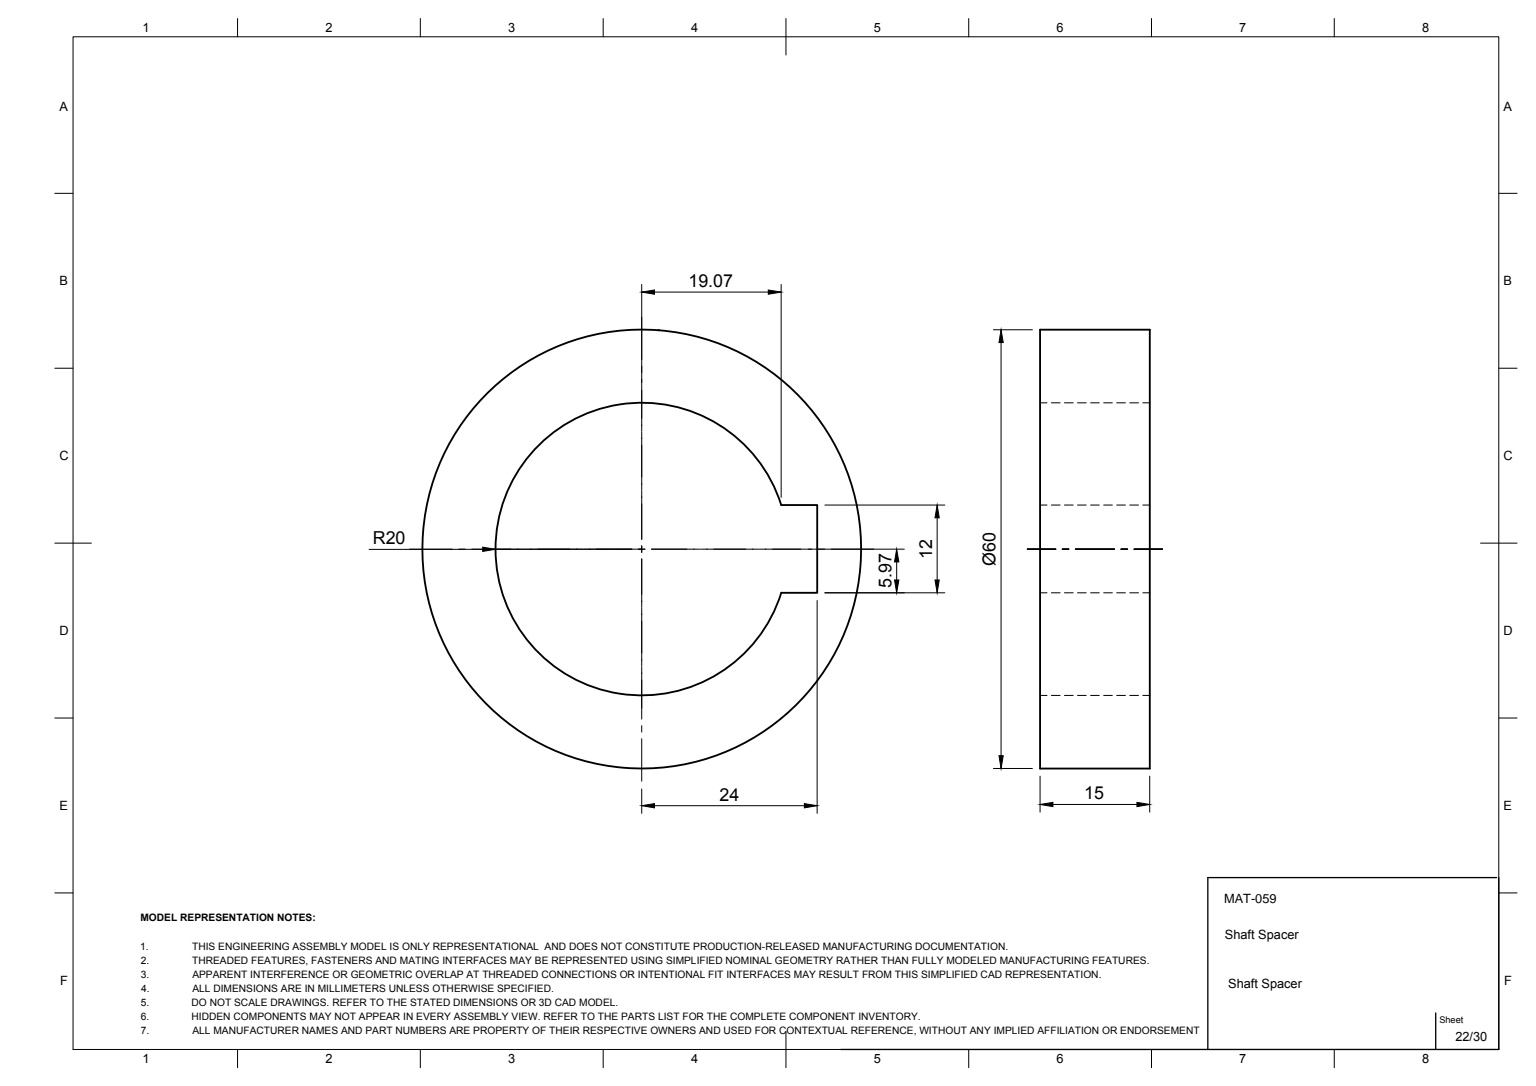
ISO-10303-21;
HEADER;
/* Generated by software containing ST-Developer
 * from STEP Tools, Inc. (www.steptools.com) 
 */

FILE_DESCRIPTION(
/* description */ ('', 'CAx-IF Rec.Pracs.---Representation and Presentation of Product Manufa
cturing Information (PMI)---4.0---2014-10-13'),
/* implementation_level */ '2;1');

FILE_NAME(
/* name */ 'Shaft Spacer.step',
/* time_stamp */ '2026-10-28T23:00:48+01:00',
/* author */ (''),
/* organization */ (''),
/* preprocessor_version */ 'ST-DEVELOPER v20.2',
/* originating_system */ 'Autodesk Translation Framework v15.17.0.0',
/* authorisation */ '');

FILE_SCHEMA (('AP242_MANAGED_MODEL_BASED_3D_ENGINEERING_MIM_LF { 1 0 10303 442 2 1 4 }'));
ENDSEC;

DATA;
#10=MECHANICAL_DESIGN_GEOMETRIC_PRESENTATION_REPRESENTATION('',(#994),#61811);
#930=SHAPE_REPRESENTATION_RELATIONSHIP('SRR','None',#61990,#955);
#955=ADVANCED_BREP_SHAPE_REPRESENTATION('',(#1033),#61803);
#994=STYLED_ITEM('',(#62156),#1033);
#1033=MANIFOLD_SOLID_BREP('Body1',#33824);
#1391=CYLINDRICAL_SURFACE('',#36117,20.);
#1392=CYLINDRICAL_SURFACE('',#36119,30.);
#2127=FACE_BOUND('',#7392,.T.);
#2128=FACE_BOUND('',#7396,.T.);
#3117=CIRCLE('',#36115,30.);
#3118=CIRCLE('',#36116,20.);
#3119=CIRCLE('',#36118,20.);
#3120=CIRCLE('',#36120,30.);
#5261=FACE_OUTER_BOUND('',#7388,.T.);
#5262=FACE_OUTER_BOUND('',#7389,.T.);
#5263=FACE_OUTER_BOUND('',#7390,.T.);
#5264=FACE_OUTER_BOUND('',#7391,.T.);
#5265=FACE_OUTER_BOUND('',#7393,.T.);
#5266=FACE_OUTER_BOUND('',#7394,.T.);
#5267=FACE_OUTER_BOUND('',#7395,.T.);
#7388=EDGE_LOOP('',(#26536,#26537,#26538,#26539));
#7389=EDGE_LOOP('',(#26540,#26541,#26542,#26543));
#7390=EDGE_LOOP('',(#26544,#26545,#26546,#26547));
#7391=EDGE_LOOP('',(#26548));
#7392=EDGE_LOOP('',(#26549,#26550,#26551,#26552));
#7393=EDGE_LOOP('',(#26553,#26554,#26555,#26556));
#7394=EDGE_LOOP('',(#26557,#26558,#26559,#26560));
#7395=EDGE_LOOP('',(#26561));
#7396=EDGE_LOOP('',(#26562,#26563,#26564,#26565));
#9813=LINE('',#56343,#12360);
#9814=LINE('',#56345,#12361);
#9815=LINE('',#56347,#12362);
#9816=LINE('',#56348,#12363);
#9817=LINE('',#56351,#12364);
#9818=LINE('',#56353,#12365);
#9819=LINE('',#56354,#12366);
#9820=LINE('',#56358,#12367);
#9821=LINE('',#56359,#12368);
#9822=LINE('',#56360,#12369);
#9823=LINE('',#56370,#12370);
#12360=VECTOR('',#43633,10.);
#12361=VECTOR('',#43634,10.);
#12362=VECTOR('',#43635,10.);
#12363=VECTOR('',#43636,10.);
#12364=VECTOR('',#43639,10.);
#12365=VECTOR('',#43640,10.);
#12366=VECTOR('',#43641,10.);
#12367=VECTOR('',#43644,10.);
#12368=VECTOR('',#43645,10.);
#12369=VECTOR('',#43646,10.);
#12370=VECTOR('',#43661,30.);
#15097=VERTEX_POINT('',#56341);
#15098=VERTEX_POINT('',#56342);
#15099=VERTEX_POINT('',#56344);
#15100=VERTEX_POINT('',#56346);
#15101=VERTEX_POINT('',#56350);
#15102=VERTEX_POINT('',#56352);
#15103=VERTEX_POINT('',#56356);
#15104=VERTEX_POINT('',#56357);
#15105=VERTEX_POINT('',#56362);
#15106=VERTEX_POINT('',#56368);
#19170=EDGE_CURVE('',#15097,#15098,#9813,.T.);
#19171=EDGE_CURVE('',#15099,#15097,#9814,.T.);
#19172=EDGE_CURVE('',#15099,#15100,#9815,.T.);
#19173=EDGE_CURVE('',#15098,#15100,#9816,.T.);
#19174=EDGE_CURVE('',#15101,#15099,#9817,.T.);
#19175=EDGE_CURVE('',#15101,#15102,#9818,.T.);
#19176=EDGE_CURVE('',#15100,#15102,#9819,.T.);
#19177=EDGE_CURVE('',#15103,#15104,#9820,.T.);
#19178=EDGE_CURVE('',#15102,#15103,#9821,.T.);
#19179=EDGE_CURVE('',#15104,#15101,#9822,.T.);
#19180=EDGE_CURVE('',#15105,#15105,#3117,.T.);
#19181=EDGE_CURVE('',#15103,#15098,#3118,.T.);
#19182=EDGE_CURVE('',#15097,#15104,#3119,.T.);
#19183=EDGE_CURVE('',#15106,#15106,#3120,.T.);
#19184=EDGE_CURVE('',#15106,#15105,#9823,.T.);
#26536=ORIENTED_EDGE('',*,*,#19170,.F.);
#26537=ORIENTED_EDGE('',*,*,#19171,.F.);
#26538=ORIENTED_EDGE('',*,*,#19172,.T.);
#26539=ORIENTED_EDGE('',*,*,#19173,.F.);
#26540=ORIENTED_EDGE('',*,*,#19174,.F.);
#26541=ORIENTED_EDGE('',*,*,#19175,.T.);
#26542=ORIENTED_EDGE('',*,*,#19176,.F.);
#26543=ORIENTED_EDGE('',*,*,#19172,.F.);
#26544=ORIENTED_EDGE('',*,*,#19177,.F.);
#26545=ORIENTED_EDGE('',*,*,#19178,.F.);
#26546=ORIENTED_EDGE('',*,*,#19175,.F.);
#26547=ORIENTED_EDGE('',*,*,#19179,.F.);
#26548=ORIENTED_EDGE('',*,*,#19180,.T.);
#26549=ORIENTED_EDGE('',*,*,#19173,.T.);
#26550=ORIENTED_EDGE('',*,*,#19176,.T.);
#26551=ORIENTED_EDGE('',*,*,#19178,.T.);
#26552=ORIENTED_EDGE('',*,*,#19181,.T.);
#26553=ORIENTED_EDGE('',*,*,#19170,.T.);
#26554=ORIENTED_EDGE('',*,*,#19181,.F.);
#26555=ORIENTED_EDGE('',*,*,#19177,.T.);
#26556=ORIENTED_EDGE('',*,*,#19182,.F.);
#26557=ORIENTED_EDGE('',*,*,#19183,.F.);
#26558=ORIENTED_EDGE('',*,*,#19184,.T.);
#26559=ORIENTED_EDGE('',*,*,#19180,.F.);
#26560=ORIENTED_EDGE('',*,*,#19184,.F.);
#26561=ORIENTED_EDGE('',*,*,#19183,.T.);
#26562=ORIENTED_EDGE('',*,*,#19171,.T.);
#26563=ORIENTED_EDGE('',*,*,#19182,.T.);
#26564=ORIENTED_EDGE('',*,*,#19179,.T.);
#26565=ORIENTED_EDGE('',*,*,#19174,.T.);
#31650=PLANE('',#36111);
#31651=PLANE('',#36112);
#31652=PLANE('',#36113);
#31653=PLANE('',#36114);
#31654=PLANE('',#36121);
#32942=ADVANCED_FACE('',(#5261),#31650,.F.);
#32943=ADVANCED_FACE('',(#5262),#31651,.F.);
#32944=ADVANCED_FACE('',(#5263),#31652,.F.);
#32945=ADVANCED_FACE('',(#5264,#2127),#31653,.T.);
#32946=ADVANCED_FACE('',(#5265),#1391,.F.);
#32947=ADVANCED_FACE('',(#5266),#1392,.T.);
#32948=ADVANCED_FACE('',(#5267,#2128),#31654,.F.);
#33824=CLOSED_SHELL('',(#32942,#32943,#32944,#32945,#32946,#32947,#32948));
#36110=AXIS2_PLACEMENT_3D('',#56339,#43629,#43630);
#36111=AXIS2_PLACEMENT_3D('',#56340,#43631,#43632);
#36112=AXIS2_PLACEMENT_3D('',#56349,#43637,#43638);
#36113=AXIS2_PLACEMENT_3D('',#56355,#43642,#43643);
#36114=AXIS2_PLACEMENT_3D('',#56361,#43647,#43648);
#36115=AXIS2_PLACEMENT_3D('',#56363,#43649,#43650);
#36116=AXIS2_PLACEMENT_3D('',#56364,#43651,#43652);
#36117=AXIS2_PLACEMENT_3D('',#56365,#43653,#43654);
#36118=AXIS2_PLACEMENT_3D('',#56366,#43655,#43656);
#36119=AXIS2_PLACEMENT_3D('',#56367,#43657,#43658);
#36120=AXIS2_PLACEMENT_3D('',#56369,#43659,#43660);
#36121=AXIS2_PLACEMENT_3D('',#56371,#43662,#43663);
#43629=DIRECTION('axis',(0.,0.,1.));
#43630=DIRECTION('refdir',(1.,0.,0.));
#43631=DIRECTION('center_axis',(-0.996957691137886,1.38453029710175E-15,
-0.0779446090567869));
#43632=DIRECTION('ref_axis',(-0.0779446090567869,-2.95972462712666E-15,
0.996957691137886));
#43633=DIRECTION('',(1.14962354933188E-15,1.,3.05863690339901E-15));
#43634=DIRECTION('',(-0.0779446090567869,-2.95972462712666E-15,0.996957691137886));
#43635=DIRECTION('',(1.14962354933188E-15,1.,3.05863690339901E-15));
#43636=DIRECTION('',(0.0779446090567869,2.95972462712666E-15,-0.996957691137886));
#43637=DIRECTION('center_axis',(0.0779446090567869,2.95972462712666E-15,
-0.996957691137886));
#43638=DIRECTION('ref_axis',(-0.996957691137886,1.38453029710175E-15,-0.0779446090567869));
#43639=DIRECTION('',(-0.996957691137886,1.38453029710175E-15,-0.0779446090567869));
#43640=DIRECTION('',(1.14962354933188E-15,1.,3.05863690339901E-15));
#43641=DIRECTION('',(0.996957691137886,-1.38453029710175E-15,0.0779446090567869));
#43642=DIRECTION('center_axis',(0.996957691137886,-1.38453029710175E-15,
0.0779446090567869));
#43643=DIRECTION('ref_axis',(0.0779446090567869,2.95972462712666E-15,-0.996957691137886));
#43644=DIRECTION('',(-1.14962354933188E-15,-1.,-3.05863690339901E-15));
#43645=DIRECTION('',(-0.0779446090567869,-2.95972462712666E-15,0.996957691137886));
#43646=DIRECTION('',(0.0779446090567869,2.95972462712666E-15,-0.996957691137886));
#43647=DIRECTION('center_axis',(1.14962354933188E-15,1.,3.05863690339901E-15));
#43648=DIRECTION('ref_axis',(0.996957691137886,-1.38453029710175E-15,0.0779446090567869));
#43649=DIRECTION('center_axis',(1.14962354933188E-15,1.,3.05863690339901E-15));
#43650=DIRECTION('ref_axis',(0.996957691137886,-1.38453029710175E-15,0.077944609056787));
#43651=DIRECTION('center_axis',(-1.14962354933188E-15,-1.,-3.05863690339901E-15));
#43652=DIRECTION('ref_axis',(0.996957691137886,-1.38453029710175E-15,0.077944609056787));
#43653=DIRECTION('center_axis',(-1.14962354933188E-15,-1.,-3.05863690339901E-15));
#43654=DIRECTION('ref_axis',(-0.079454779543177,-2.95762384959718E-15,0.99683847137224));
#43655=DIRECTION('center_axis',(1.14962354933188E-15,1.,3.05863690339901E-15));
#43656=DIRECTION('ref_axis',(0.996957691137886,-1.38453029710175E-15,0.077944609056787));
#43657=DIRECTION('center_axis',(-1.14962354933188E-15,-1.,-3.05863690339901E-15));
#43658=DIRECTION('ref_axis',(0.996957691137886,-1.38453029710175E-15,0.077944609056787));
#43659=DIRECTION('center_axis',(-1.14962354933188E-15,-1.,-3.05863690339901E-15));
#43660=DIRECTION('ref_axis',(0.996957691137886,-1.38453029710175E-15,0.077944609056787));
#43661=DIRECTION('',(1.14962354933188E-15,1.,3.05863690339901E-15));
#43662=DIRECTION('center_axis',(1.14962354933188E-15,1.,3.05863690339901E-15));
#43663=DIRECTION('ref_axis',(0.996957691137886,-1.38453029710175E-15,0.0779446090567869));
#56339=CARTESIAN_POINT('',(0.,0.,0.));
#56340=CARTESIAN_POINT('Origin',(371.018259814925,-255.47200726879,420.650814731371));
#56341=CARTESIAN_POINT('',(370.635385768447,-255.47200726879,425.548000437897));
#56342=CARTESIAN_POINT('',(370.635385768447,-240.47200726879,425.548000437897));
#56343=CARTESIAN_POINT('',(370.635385768447,-240.47200726879,425.548000437897));
#56344=CARTESIAN_POINT('',(371.018259814925,-255.47200726879,420.650814731371));
#56345=CARTESIAN_POINT('',(370.082925320099,-255.47200726879,432.614296615326));
#56346=CARTESIAN_POINT('',(371.018259814925,-240.47200726879,420.650814731371));
#56347=CARTESIAN_POINT('',(371.018259814925,-255.47200726879,420.650814731371));
#56348=CARTESIAN_POINT('',(370.082925320099,-240.47200726879,432.614296615326));
#56349=CARTESIAN_POINT('Origin',(382.98175210858,-255.47200726879,421.586150040052));
#56350=CARTESIAN_POINT('',(382.98175210858,-255.47200726879,421.586150040052));
#56351=CARTESIAN_POINT('',(379.97647207537,-255.47200726879,421.351189841262));
#56352=CARTESIAN_POINT('',(382.98175210858,-240.47200726879,421.586150040052));
#56353=CARTESIAN_POINT('',(382.98175210858,-255.47200726879,421.586150040052));
#56354=CARTESIAN_POINT('',(379.97647207537,-240.47200726879,421.351189841262));
#56355=CARTESIAN_POINT('Origin',(382.358195236125,-255.47200726879,429.561811569155));
#56356=CARTESIAN_POINT('',(382.597461150368,-240.47200726879,426.501458886426));
#56357=CARTESIAN_POINT('',(382.597461150368,-255.47200726879,426.501458886426));
#56358=CARTESIAN_POINT('',(382.597461150368,-240.47200726879,426.501458886426));
#56359=CARTESIAN_POINT('',(381.734639177527,-240.47200726879,437.537462688559));
#56360=CARTESIAN_POINT('',(381.734639177527,-255.47200726879,437.537462688559));
#56361=CARTESIAN_POINT('Origin',(375.100523052509,-240.47200726879,445.043193410383));
#56362=CARTESIAN_POINT('',(345.191792318373,-240.47200726879,442.704855138679));
#56363=CARTESIAN_POINT('Origin',(375.100523052509,-240.47200726879,445.043193410383));
#56364=CARTESIAN_POINT('Origin',(375.100523052509,-240.47200726879,445.043193410383));
#56365=CARTESIAN_POINT('Origin',(375.100523052509,-240.47200726879,445.043193410383));
#56366=CARTESIAN_POINT('Origin',(375.100523052509,-255.47200726879,445.043193410383));
#56367=CARTESIAN_POINT('Origin',(375.100523052509,-240.47200726879,445.043193410383));
#56368=CARTESIAN_POINT('',(345.191792318373,-255.47200726879,442.704855138679));
#56369=CARTESIAN_POINT('Origin',(375.100523052509,-255.47200726879,445.043193410383));
#56370=CARTESIAN_POINT('',(345.191792318373,-240.47200726879,442.704855138679));
#56371=CARTESIAN_POINT('Origin',(375.100523052509,-255.47200726879,445.043193410383));
#61772=UNCERTAINTY_MEASURE_WITH_UNIT(LENGTH_MEASURE(0.01),#61812,
'DISTANCE_ACCURACY_VALUE',
'Maximum model space distance between geometric entities at asserted c
onnectivities');
#61780=UNCERTAINTY_MEASURE_WITH_UNIT(LENGTH_MEASURE(0.01),#61812,
'DISTANCE_ACCURACY_VALUE',
'Maximum model space distance between geometric entities at asserted c
onnectivities');
#61803=(
GEOMETRIC_REPRESENTATION_CONTEXT(3)
GLOBAL_UNCERTAINTY_ASSIGNED_CONTEXT((#61772))
GLOBAL_UNIT_ASSIGNED_CONTEXT((#61812,#61814,#61815))
REPRESENTATION_CONTEXT('','3D')
);
#61811=(
GEOMETRIC_REPRESENTATION_CONTEXT(3)
GLOBAL_UNCERTAINTY_ASSIGNED_CONTEXT((#61780))
GLOBAL_UNIT_ASSIGNED_CONTEXT((#61812,#61814,#61815))
REPRESENTATION_CONTEXT('','3D')
);
#61812=(
LENGTH_UNIT()
NAMED_UNIT(*)
SI_UNIT(.MILLI.,.METRE.)
);
#61814=(
NAMED_UNIT(*)
PLANE_ANGLE_UNIT()
SI_UNIT($,.RADIAN.)
);
#61815=(
NAMED_UNIT(*)
SI_UNIT($,.STERADIAN.)
SOLID_ANGLE_UNIT()
);
#61838=SHAPE_DEFINITION_REPRESENTATION(#61884,#61990);
#61884=PRODUCT_DEFINITION_SHAPE('',$,#62021);
#61990=SHAPE_REPRESENTATION('',(#36110),#61803);
#61998=PRODUCT_DEFINITION_CONTEXT('part definition',#62090,'design');
#62021=PRODUCT_DEFINITION('Shaft Spacer','Shaft Spacer',#62051,#61998);
#62051=PRODUCT_DEFINITION_FORMATION('',$,#62114);
#62090=APPLICATION_CONTEXT('Managed model based 3d engineering');
#62091=PRODUCT_CONTEXT('part definition',#62090,'mechanical');
#62114=PRODUCT('Shaft Spacer','Shaft Spacer',$,(#62091));
#62150=COLOUR_RGB('Grey',0.48,0.52,0.57);
#62151=FILL_AREA_STYLE_COLOUR('',#62150);
#62152=FILL_AREA_STYLE('',(#62151));
#62153=SURFACE_STYLE_FILL_AREA(#62152);
#62154=SURFACE_SIDE_STYLE('',(#62153));
#62155=SURFACE_STYLE_USAGE(.BOTH.,#62154);
#62156=PRESENTATION_STYLE_ASSIGNMENT((#62155));
ENDSEC;
END-ISO-10303-21;
